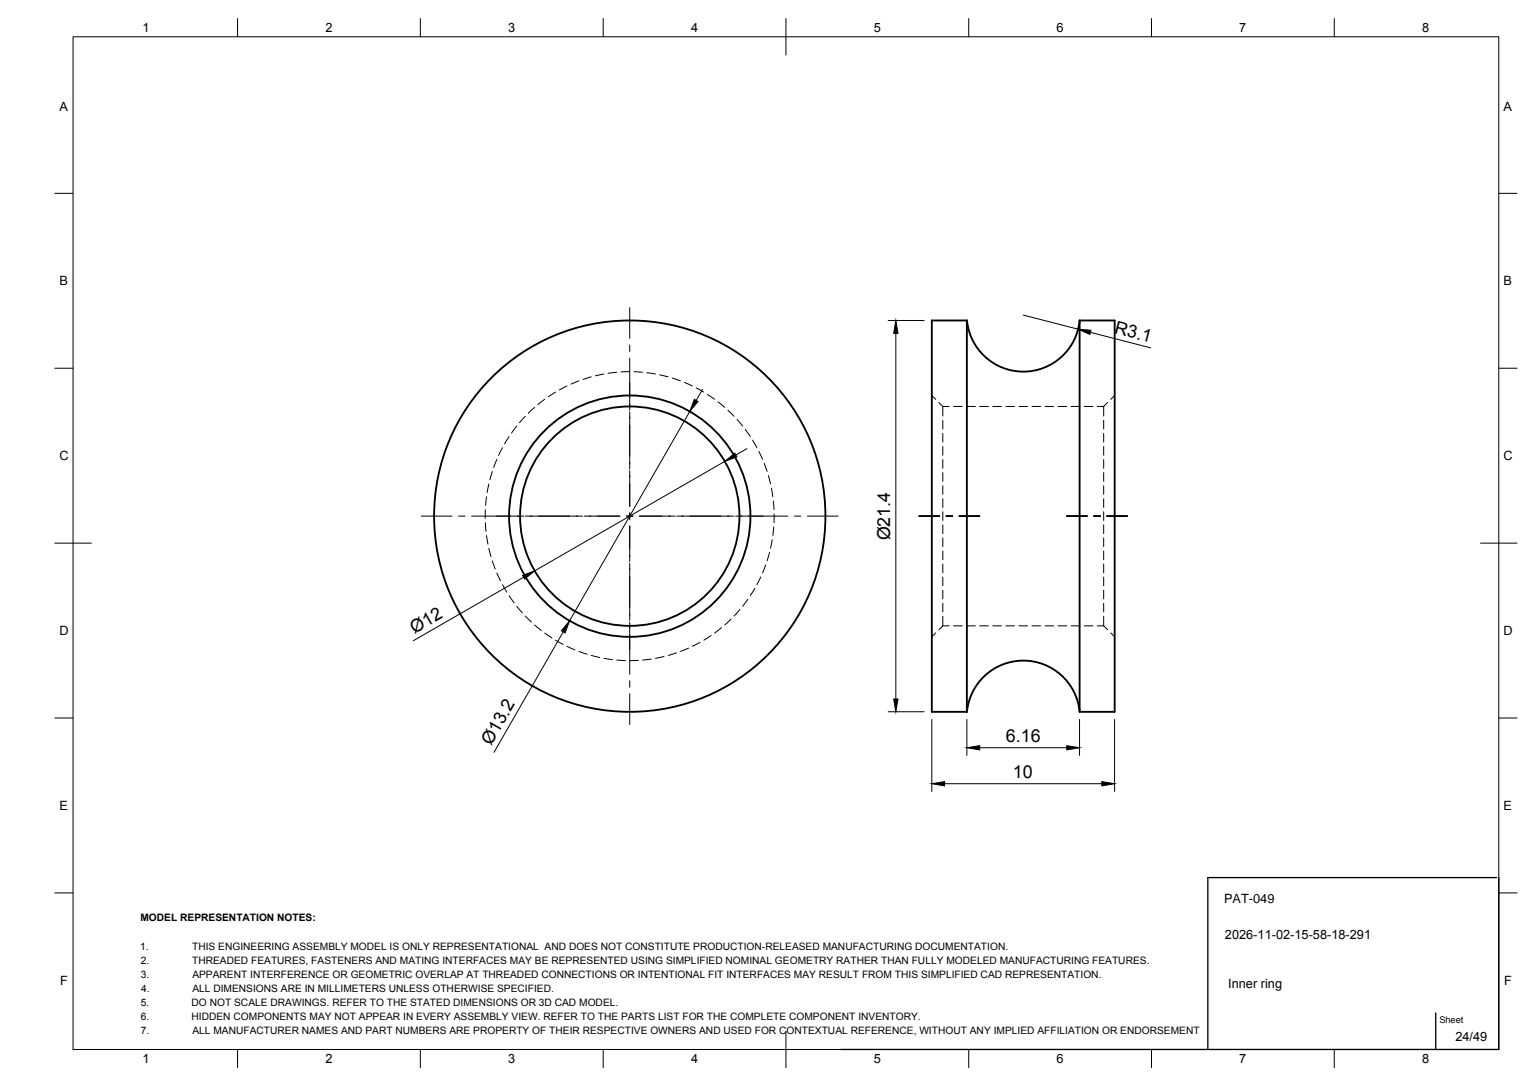
ISO-10303-21;
HEADER;
/* Generated by software containing ST-Developer
 * from STEP Tools, Inc. (www.steptools.com) 
 */

FILE_DESCRIPTION(
/* description */ ('Hand drill press frame (manual)'),
/* implementation_level */ '2;1');

FILE_NAME(
/* name */ 'Inner ring.step',
/* time_stamp */ '2026-10-28T03:25:28-07:00',
/* author */ (''),
/* organization */ (''),
/* preprocessor_version */ 'ST-DEVELOPER v20.2',
/* originating_system */ 'Autodesk Translation Framework v15.17.0.0',
/* authorisation */ '');

FILE_SCHEMA (('AUTOMOTIVE_DESIGN { 1 0 10303 214 3 1 1 }'));
ENDSEC;

DATA;
#10=MECHANICAL_DESIGN_GEOMETRIC_PRESENTATION_REPRESENTATION('',(#636),#33299);
#471=TOROIDAL_SURFACE('',#13605,1.1,0.309556);
#474=CONICAL_SURFACE('',#13616,0.63,0.785398163397448);
#475=CONICAL_SURFACE('',#13623,0.63,0.785398163397448);
#546=SHAPE_REPRESENTATION_RELATIONSHIP('SRR','None',#33506,#591);
#591=ADVANCED_BREP_SHAPE_REPRESENTATION('',(#688),#33268);
#636=STYLED_ITEM('',(#33814),#688);
#688=MANIFOLD_SOLID_BREP('Body1',#12654);
#836=FACE_BOUND('',#2366,.T.);
#837=FACE_BOUND('',#2369,.T.);
#1017=PLANE('',#13618);
#1018=PLANE('',#13621);
#1556=FACE_OUTER_BOUND('',#2361,.T.);
#1557=FACE_OUTER_BOUND('',#2362,.T.);
#1558=FACE_OUTER_BOUND('',#2363,.T.);
#1559=FACE_OUTER_BOUND('',#2364,.T.);
#1560=FACE_OUTER_BOUND('',#2365,.T.);
#1561=FACE_OUTER_BOUND('',#2367,.T.);
#1562=FACE_OUTER_BOUND('',#2368,.T.);
#1563=FACE_OUTER_BOUND('',#2370,.T.);
#2361=EDGE_LOOP('',(#9447,#9448,#9449,#9450,#9451,#9452));
#2362=EDGE_LOOP('',(#9453,#9454,#9455,#9456,#9457));
#2363=EDGE_LOOP('',(#9458,#9459,#9460,#9461));
#2364=EDGE_LOOP('',(#9462,#9463,#9464,#9465));
#2365=EDGE_LOOP('',(#9466));
#2366=EDGE_LOOP('',(#9467));
#2367=EDGE_LOOP('',(#9468,#9469,#9470,#9471,#9472));
#2368=EDGE_LOOP('',(#9473));
#2369=EDGE_LOOP('',(#9474));
#2370=EDGE_LOOP('',(#9475,#9476,#9477,#9478));
#3203=LINE('',#19178,#4368);
#3204=LINE('',#19184,#4369);
#3205=LINE('',#19188,#4370);
#3206=LINE('',#19194,#4371);
#3207=LINE('',#19199,#4372);
#4368=VECTOR('',#15534,1.070235);
#4369=VECTOR('',#15541,0.6);
#4370=VECTOR('',#15546,0.63);
#4371=VECTOR('',#15555,1.070235);
#4372=VECTOR('',#15562,0.63);
#5393=CIRCLE('',#13606,1.070235);
#5394=CIRCLE('',#13607,1.070235);
#5395=CIRCLE('',#13608,0.309556);
#5396=CIRCLE('',#13609,1.070235);
#5397=CIRCLE('',#13610,1.070235);
#5398=CIRCLE('',#13612,1.070235);
#5399=CIRCLE('',#13614,0.6);
#5400=CIRCLE('',#13615,0.6);
#5401=CIRCLE('',#13617,0.66);
#5402=CIRCLE('',#13620,1.070235);
#5403=CIRCLE('',#13622,0.66);
#5955=VERTEX_POINT('',#19167);
#5956=VERTEX_POINT('',#19168);
#5957=VERTEX_POINT('',#19171);
#5958=VERTEX_POINT('',#19173);
#5959=VERTEX_POINT('',#19177);
#5960=VERTEX_POINT('',#19181);
#5961=VERTEX_POINT('',#19183);
#5962=VERTEX_POINT('',#19187);
#5963=VERTEX_POINT('',#19192);
#5964=VERTEX_POINT('',#19196);
#7252=EDGE_CURVE('',#5955,#5956,#5393,.T.);
#7253=EDGE_CURVE('',#5956,#5955,#5394,.T.);
#7254=EDGE_CURVE('',#5956,#5957,#5395,.T.);
#7255=EDGE_CURVE('',#5958,#5957,#5396,.T.);
#7256=EDGE_CURVE('',#5957,#5958,#5397,.T.);
#7257=EDGE_CURVE('',#5958,#5959,#3203,.T.);
#7258=EDGE_CURVE('',#5959,#5959,#5398,.T.);
#7259=EDGE_CURVE('',#5960,#5960,#5399,.T.);
#7260=EDGE_CURVE('',#5960,#5961,#3204,.T.);
#7261=EDGE_CURVE('',#5961,#5961,#5400,.T.);
#7262=EDGE_CURVE('',#5961,#5962,#3205,.T.);
#7263=EDGE_CURVE('',#5962,#5962,#5401,.T.);
#7264=EDGE_CURVE('',#5963,#5963,#5402,.T.);
#7265=EDGE_CURVE('',#5963,#5955,#3206,.T.);
#7266=EDGE_CURVE('',#5964,#5964,#5403,.T.);
#7267=EDGE_CURVE('',#5964,#5960,#3207,.T.);
#9447=ORIENTED_EDGE('',*,*,#7252,.F.);
#9448=ORIENTED_EDGE('',*,*,#7253,.F.);
#9449=ORIENTED_EDGE('',*,*,#7254,.T.);
#9450=ORIENTED_EDGE('',*,*,#7255,.F.);
#9451=ORIENTED_EDGE('',*,*,#7256,.F.);
#9452=ORIENTED_EDGE('',*,*,#7254,.F.);
#9453=ORIENTED_EDGE('',*,*,#7255,.T.);
#9454=ORIENTED_EDGE('',*,*,#7256,.T.);
#9455=ORIENTED_EDGE('',*,*,#7257,.T.);
#9456=ORIENTED_EDGE('',*,*,#7258,.T.);
#9457=ORIENTED_EDGE('',*,*,#7257,.F.);
#9458=ORIENTED_EDGE('',*,*,#7259,.T.);
#9459=ORIENTED_EDGE('',*,*,#7260,.T.);
#9460=ORIENTED_EDGE('',*,*,#7261,.F.);
#9461=ORIENTED_EDGE('',*,*,#7260,.F.);
#9462=ORIENTED_EDGE('',*,*,#7261,.T.);
#9463=ORIENTED_EDGE('',*,*,#7262,.T.);
#9464=ORIENTED_EDGE('',*,*,#7263,.F.);
#9465=ORIENTED_EDGE('',*,*,#7262,.F.);
#9466=ORIENTED_EDGE('',*,*,#7258,.F.);
#9467=ORIENTED_EDGE('',*,*,#7263,.T.);
#9468=ORIENTED_EDGE('',*,*,#7264,.F.);
#9469=ORIENTED_EDGE('',*,*,#7265,.T.);
#9470=ORIENTED_EDGE('',*,*,#7252,.T.);
#9471=ORIENTED_EDGE('',*,*,#7253,.T.);
#9472=ORIENTED_EDGE('',*,*,#7265,.F.);
#9473=ORIENTED_EDGE('',*,*,#7264,.T.);
#9474=ORIENTED_EDGE('',*,*,#7266,.F.);
#9475=ORIENTED_EDGE('',*,*,#7266,.T.);
#9476=ORIENTED_EDGE('',*,*,#7267,.T.);
#9477=ORIENTED_EDGE('',*,*,#7259,.F.);
#9478=ORIENTED_EDGE('',*,*,#7267,.F.);
#11871=CYLINDRICAL_SURFACE('',#13611,1.070235);
#11872=CYLINDRICAL_SURFACE('',#13613,0.6);
#11873=CYLINDRICAL_SURFACE('',#13619,1.070235);
#12165=ADVANCED_FACE('',(#1556),#471,.F.);
#12166=ADVANCED_FACE('',(#1557),#11871,.T.);
#12167=ADVANCED_FACE('',(#1558),#11872,.F.);
#12168=ADVANCED_FACE('',(#1559),#474,.F.);
#12169=ADVANCED_FACE('',(#1560,#836),#1017,.T.);
#12170=ADVANCED_FACE('',(#1561),#11873,.T.);
#12171=ADVANCED_FACE('',(#1562,#837),#1018,.T.);
#12172=ADVANCED_FACE('',(#1563),#475,.F.);
#12654=CLOSED_SHELL('',(#12165,#12166,#12167,#12168,#12169,#12170,#12171,
#12172));
#13604=AXIS2_PLACEMENT_3D('',#19165,#15518,#15519);
#13605=AXIS2_PLACEMENT_3D('',#19166,#15520,#15521);
#13606=AXIS2_PLACEMENT_3D('',#19169,#15522,#15523);
#13607=AXIS2_PLACEMENT_3D('',#19170,#15524,#15525);
#13608=AXIS2_PLACEMENT_3D('',#19172,#15526,#15527);
#13609=AXIS2_PLACEMENT_3D('',#19174,#15528,#15529);
#13610=AXIS2_PLACEMENT_3D('',#19175,#15530,#15531);
#13611=AXIS2_PLACEMENT_3D('',#19176,#15532,#15533);
#13612=AXIS2_PLACEMENT_3D('',#19179,#15535,#15536);
#13613=AXIS2_PLACEMENT_3D('',#19180,#15537,#15538);
#13614=AXIS2_PLACEMENT_3D('',#19182,#15539,#15540);
#13615=AXIS2_PLACEMENT_3D('',#19185,#15542,#15543);
#13616=AXIS2_PLACEMENT_3D('',#19186,#15544,#15545);
#13617=AXIS2_PLACEMENT_3D('',#19189,#15547,#15548);
#13618=AXIS2_PLACEMENT_3D('',#19190,#15549,#15550);
#13619=AXIS2_PLACEMENT_3D('',#19191,#15551,#15552);
#13620=AXIS2_PLACEMENT_3D('',#19193,#15553,#15554);
#13621=AXIS2_PLACEMENT_3D('',#19195,#15556,#15557);
#13622=AXIS2_PLACEMENT_3D('',#19197,#15558,#15559);
#13623=AXIS2_PLACEMENT_3D('',#19198,#15560,#15561);
#15518=DIRECTION('axis',(0.,0.,1.));
#15519=DIRECTION('refdir',(1.,0.,0.));
#15520=DIRECTION('center_axis',(0.,-1.,0.));
#15521=DIRECTION('ref_axis',(0.,0.,-1.));
#15522=DIRECTION('center_axis',(0.,-1.,0.));
#15523=DIRECTION('ref_axis',(1.,0.,0.));
#15524=DIRECTION('center_axis',(0.,-1.,0.));
#15525=DIRECTION('ref_axis',(1.,0.,0.));
#15526=DIRECTION('center_axis',(1.,0.,1.22464679914735E-16));
#15527=DIRECTION('ref_axis',(-1.22464679914735E-16,0.,1.));
#15528=DIRECTION('center_axis',(0.,1.,0.));
#15529=DIRECTION('ref_axis',(1.,0.,0.));
#15530=DIRECTION('center_axis',(0.,1.,0.));
#15531=DIRECTION('ref_axis',(1.,0.,0.));
#15532=DIRECTION('center_axis',(0.,-1.,0.));
#15533=DIRECTION('ref_axis',(1.,0.,0.));
#15534=DIRECTION('',(0.,1.,0.));
#15535=DIRECTION('center_axis',(0.,-1.,0.));
#15536=DIRECTION('ref_axis',(1.,0.,0.));
#15537=DIRECTION('center_axis',(0.,-1.,0.));
#15538=DIRECTION('ref_axis',(1.,0.,0.));
#15539=DIRECTION('center_axis',(0.,-1.,0.));
#15540=DIRECTION('ref_axis',(1.,0.,0.));
#15541=DIRECTION('',(0.,1.,0.));
#15542=DIRECTION('center_axis',(0.,-1.,0.));
#15543=DIRECTION('ref_axis',(1.,0.,0.));
#15544=DIRECTION('center_axis',(0.,1.,0.));
#15545=DIRECTION('ref_axis',(1.,0.,0.));
#15546=DIRECTION('',(-0.707106781186548,0.707106781186547,-8.65956056235493E-17));
#15547=DIRECTION('center_axis',(0.,-1.,0.));
#15548=DIRECTION('ref_axis',(1.,0.,0.));
#15549=DIRECTION('center_axis',(0.,1.,0.));
#15550=DIRECTION('ref_axis',(0.,0.,1.));
#15551=DIRECTION('center_axis',(0.,-1.,0.));
#15552=DIRECTION('ref_axis',(1.,0.,0.));
#15553=DIRECTION('center_axis',(0.,-1.,0.));
#15554=DIRECTION('ref_axis',(1.,0.,0.));
#15555=DIRECTION('',(0.,1.,0.));
#15556=DIRECTION('center_axis',(0.,-1.,0.));
#15557=DIRECTION('ref_axis',(0.,0.,-1.));
#15558=DIRECTION('center_axis',(0.,-1.,0.));
#15559=DIRECTION('ref_axis',(1.,0.,0.));
#15560=DIRECTION('center_axis',(0.,-1.,0.));
#15561=DIRECTION('ref_axis',(1.,0.,0.));
#15562=DIRECTION('',(0.707106781186548,0.707106781186547,8.65956056235493E-17));
#19165=CARTESIAN_POINT('',(0.,0.,0.));
#19166=CARTESIAN_POINT('Origin',(0.,0.,0.));
#19167=CARTESIAN_POINT('',(-1.070235,-0.308121667383195,-1.31065986708547E-16));
#19168=CARTESIAN_POINT('',(-1.31065986708547E-16,-0.308121667383195,1.070235));
#19169=CARTESIAN_POINT('Origin',(0.,-0.308121667383195,0.));
#19170=CARTESIAN_POINT('Origin',(0.,-0.308121667383195,0.));
#19171=CARTESIAN_POINT('',(-1.31065986708547E-16,0.308121667383195,1.070235));
#19172=CARTESIAN_POINT('Origin',(-1.34711147906209E-16,0.,1.1));
#19173=CARTESIAN_POINT('',(-1.070235,0.308121667383195,1.31065986708547E-16));
#19174=CARTESIAN_POINT('Origin',(0.,0.308121667383195,0.));
#19175=CARTESIAN_POINT('Origin',(0.,0.308121667383195,0.));
#19176=CARTESIAN_POINT('Origin',(0.,0.,0.));
#19177=CARTESIAN_POINT('',(-1.070235,0.5,-1.31065986708547E-16));
#19178=CARTESIAN_POINT('',(-1.070235,0.,-1.31065986708547E-16));
#19179=CARTESIAN_POINT('Origin',(0.,0.5,0.));
#19180=CARTESIAN_POINT('Origin',(0.,0.,0.));
#19181=CARTESIAN_POINT('',(-0.6,-0.44,-7.34788079488412E-17));
#19182=CARTESIAN_POINT('Origin',(0.,-0.44,0.));
#19183=CARTESIAN_POINT('',(-0.6,0.44,-7.34788079488412E-17));
#19184=CARTESIAN_POINT('',(-0.6,0.,-7.34788079488412E-17));
#19185=CARTESIAN_POINT('Origin',(0.,0.44,0.));
#19186=CARTESIAN_POINT('Origin',(0.,0.47,0.));
#19187=CARTESIAN_POINT('',(-0.66,0.5,-8.08266887437253E-17));
#19188=CARTESIAN_POINT('',(-0.63,0.47,-7.71527483462832E-17));
#19189=CARTESIAN_POINT('Origin',(0.,0.5,0.));
#19190=CARTESIAN_POINT('Origin',(1.070235,0.5,0.));
#19191=CARTESIAN_POINT('Origin',(0.,0.,0.));
#19192=CARTESIAN_POINT('',(-1.070235,-0.5,-1.31065986708547E-16));
#19193=CARTESIAN_POINT('Origin',(0.,-0.5,0.));
#19194=CARTESIAN_POINT('',(-1.070235,0.,-1.31065986708547E-16));
#19195=CARTESIAN_POINT('Origin',(0.66,-0.5,0.));
#19196=CARTESIAN_POINT('',(-0.66,-0.5,-8.08266887437253E-17));
#19197=CARTESIAN_POINT('Origin',(0.,-0.5,0.));
#19198=CARTESIAN_POINT('Origin',(0.,-0.47,0.));
#19199=CARTESIAN_POINT('',(-0.63,-0.47,-7.71527483462832E-17));
#33216=UNCERTAINTY_MEASURE_WITH_UNIT(LENGTH_MEASURE(0.001),#33300,
'DISTANCE_ACCURACY_VALUE',
'Maximum model space distance between geometric entities at asserted c
onnectivities');
#33247=UNCERTAINTY_MEASURE_WITH_UNIT(LENGTH_MEASURE(0.001),#33300,
'DISTANCE_ACCURACY_VALUE',
'Maximum model space distance between geometric entities at asserted c
onnectivities');
#33268=(
GEOMETRIC_REPRESENTATION_CONTEXT(3)
GLOBAL_UNCERTAINTY_ASSIGNED_CONTEXT((#33216))
GLOBAL_UNIT_ASSIGNED_CONTEXT((#33300,#33302,#33303))
REPRESENTATION_CONTEXT('','3D')
);
#33299=(
GEOMETRIC_REPRESENTATION_CONTEXT(3)
GLOBAL_UNCERTAINTY_ASSIGNED_CONTEXT((#33247))
GLOBAL_UNIT_ASSIGNED_CONTEXT((#33300,#33302,#33303))
REPRESENTATION_CONTEXT('','3D')
);
#33300=(
LENGTH_UNIT()
NAMED_UNIT(*)
SI_UNIT(.CENTI.,.METRE.)
);
#33302=(
NAMED_UNIT(*)
PLANE_ANGLE_UNIT()
SI_UNIT($,.RADIAN.)
);
#33303=(
NAMED_UNIT(*)
SI_UNIT($,.STERADIAN.)
SOLID_ANGLE_UNIT()
);
#33324=SHAPE_DEFINITION_REPRESENTATION(#33375,#33506);
#33375=PRODUCT_DEFINITION_SHAPE('',$,#33558);
#33506=SHAPE_REPRESENTATION('',(#13604),#33268);
#33537=PRODUCT_DEFINITION_CONTEXT('part definition',#33692,'design');
#33558=PRODUCT_DEFINITION('Inner ring','Inner ring',#33609,#33537);
#33609=PRODUCT_DEFINITION_FORMATION('',$,#33714);
#33692=APPLICATION_CONTEXT(
'Core Data for Automotive Mechanical Design Process');
#33693=PRODUCT_CONTEXT('part definition',#33692,'mechanical');
#33714=PRODUCT('Inner ring','Inner ring','Inner ring',(#33693));
#33808=COLOUR_RGB('Grey',0.48,0.52,0.57);
#33809=FILL_AREA_STYLE_COLOUR('',#33808);
#33810=FILL_AREA_STYLE('',(#33809));
#33811=SURFACE_STYLE_FILL_AREA(#33810);
#33812=SURFACE_SIDE_STYLE('',(#33811));
#33813=SURFACE_STYLE_USAGE(.BOTH.,#33812);
#33814=PRESENTATION_STYLE_ASSIGNMENT((#33813));
ENDSEC;
END-ISO-10303-21;
